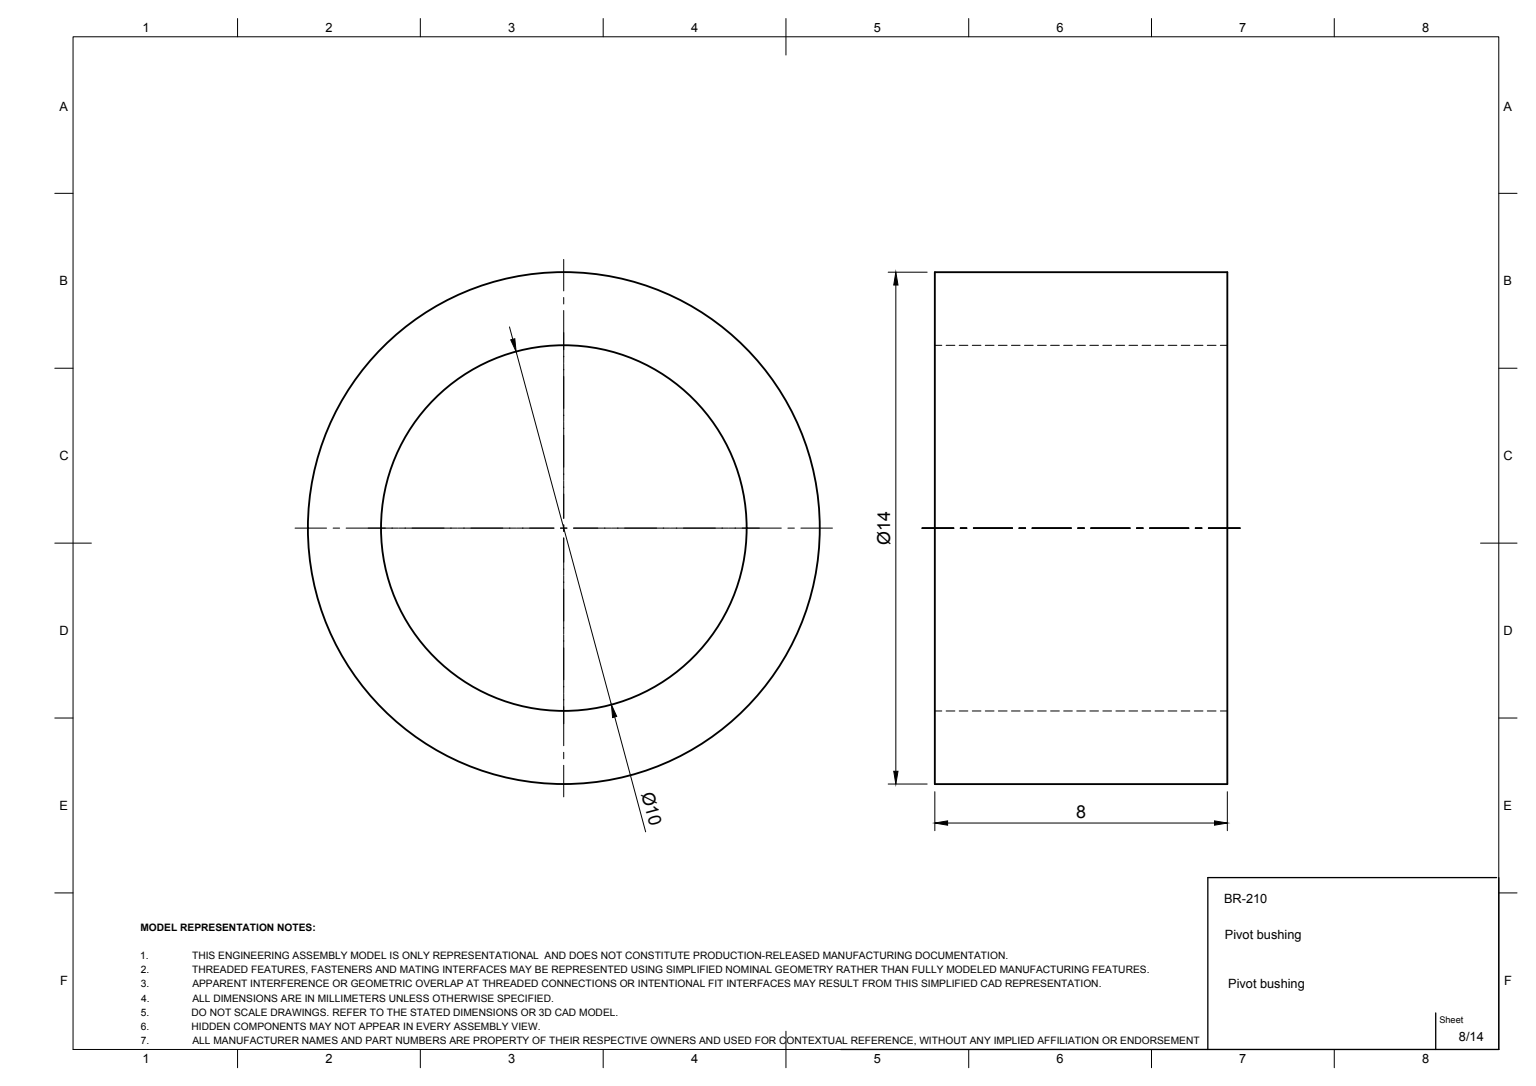
ISO-10303-21;
HEADER;
/* Generated by software containing ST-Developer
 * from STEP Tools, Inc. (www.steptools.com) 
 */

FILE_DESCRIPTION(
/* description */ ('Independent 1:2 reduction pantograph. 120 mm parallelogram sides; fix
ed fulcrum on the extension of a 240 mm link. Drawing point halfway al
ong its link, so its XY displacement is one half of the tracing point.
 Replaceable pivot bushes and retained pins. Calibration and productio
n accuracy unassigned.'),
/* implementation_level */ '2;1');

FILE_NAME(
/* name */ 'Pivot bushing.step',
/* time_stamp */ '2026-11-07T22:11:57-08:00',
/* author */ (''),
/* organization */ (''),
/* preprocessor_version */ 'ST-DEVELOPER v20.2',
/* originating_system */ 'Autodesk Translation Framework v15.17.0.0',
/* authorisation */ '');

FILE_SCHEMA (('AUTOMOTIVE_DESIGN { 1 0 10303 214 3 1 1 }'));
ENDSEC;

DATA;
#10=MECHANICAL_DESIGN_GEOMETRIC_PRESENTATION_REPRESENTATION('',(#194),#2926);
#168=SHAPE_REPRESENTATION_RELATIONSHIP('SRR','None',#3005,#181);
#181=ADVANCED_BREP_SHAPE_REPRESENTATION('',(#207),#2921);
#194=STYLED_ITEM('',(#3078),#207);
#207=MANIFOLD_SOLID_BREP('Body1',#1549);
#251=FACE_BOUND('',#505,.T.);
#252=FACE_BOUND('',#507,.T.);
#291=PLANE('',#1846);
#292=PLANE('',#1847);
#371=FACE_OUTER_BOUND('',#502,.T.);
#372=FACE_OUTER_BOUND('',#503,.T.);
#373=FACE_OUTER_BOUND('',#504,.T.);
#374=FACE_OUTER_BOUND('',#506,.T.);
#502=EDGE_LOOP('',(#1325,#1326,#1327,#1328));
#503=EDGE_LOOP('',(#1329,#1330,#1331,#1332));
#504=EDGE_LOOP('',(#1333));
#505=EDGE_LOOP('',(#1334));
#506=EDGE_LOOP('',(#1335));
#507=EDGE_LOOP('',(#1336));
#598=LINE('',#2767,#679);
#599=LINE('',#2773,#680);
#679=VECTOR('',#2280,5.);
#680=VECTOR('',#2287,7.);
#763=CIRCLE('',#1841,5.);
#764=CIRCLE('',#1842,5.);
#765=CIRCLE('',#1844,7.);
#766=CIRCLE('',#1845,7.);
#871=VERTEX_POINT('',#2764);
#872=VERTEX_POINT('',#2766);
#873=VERTEX_POINT('',#2770);
#874=VERTEX_POINT('',#2772);
#1027=EDGE_CURVE('',#871,#871,#763,.T.);
#1028=EDGE_CURVE('',#871,#872,#598,.T.);
#1029=EDGE_CURVE('',#872,#872,#764,.T.);
#1030=EDGE_CURVE('',#873,#873,#765,.T.);
#1031=EDGE_CURVE('',#873,#874,#599,.T.);
#1032=EDGE_CURVE('',#874,#874,#766,.T.);
#1325=ORIENTED_EDGE('',*,*,#1027,.F.);
#1326=ORIENTED_EDGE('',*,*,#1028,.T.);
#1327=ORIENTED_EDGE('',*,*,#1029,.T.);
#1328=ORIENTED_EDGE('',*,*,#1028,.F.);
#1329=ORIENTED_EDGE('',*,*,#1030,.F.);
#1330=ORIENTED_EDGE('',*,*,#1031,.T.);
#1331=ORIENTED_EDGE('',*,*,#1032,.T.);
#1332=ORIENTED_EDGE('',*,*,#1031,.F.);
#1333=ORIENTED_EDGE('',*,*,#1030,.T.);
#1334=ORIENTED_EDGE('',*,*,#1027,.T.);
#1335=ORIENTED_EDGE('',*,*,#1032,.F.);
#1336=ORIENTED_EDGE('',*,*,#1029,.F.);
#1438=CYLINDRICAL_SURFACE('',#1840,5.);
#1439=CYLINDRICAL_SURFACE('',#1843,7.);
#1515=ADVANCED_FACE('',(#371),#1438,.F.);
#1516=ADVANCED_FACE('',(#372),#1439,.T.);
#1517=ADVANCED_FACE('',(#373,#251),#291,.T.);
#1518=ADVANCED_FACE('',(#374,#252),#292,.F.);
#1549=CLOSED_SHELL('',(#1515,#1516,#1517,#1518));
#1839=AXIS2_PLACEMENT_3D('',#2762,#2274,#2275);
#1840=AXIS2_PLACEMENT_3D('',#2763,#2276,#2277);
#1841=AXIS2_PLACEMENT_3D('',#2765,#2278,#2279);
#1842=AXIS2_PLACEMENT_3D('',#2768,#2281,#2282);
#1843=AXIS2_PLACEMENT_3D('',#2769,#2283,#2284);
#1844=AXIS2_PLACEMENT_3D('',#2771,#2285,#2286);
#1845=AXIS2_PLACEMENT_3D('',#2774,#2288,#2289);
#1846=AXIS2_PLACEMENT_3D('',#2775,#2290,#2291);
#1847=AXIS2_PLACEMENT_3D('',#2776,#2292,#2293);
#2274=DIRECTION('axis',(0.,0.,1.));
#2275=DIRECTION('refdir',(1.,0.,0.));
#2276=DIRECTION('center_axis',(0.,0.,1.));
#2277=DIRECTION('ref_axis',(1.,0.,0.));
#2278=DIRECTION('center_axis',(0.,0.,-1.));
#2279=DIRECTION('ref_axis',(1.,0.,0.));
#2280=DIRECTION('',(0.,0.,-1.));
#2281=DIRECTION('center_axis',(0.,0.,-1.));
#2282=DIRECTION('ref_axis',(1.,0.,0.));
#2283=DIRECTION('center_axis',(0.,0.,1.));
#2284=DIRECTION('ref_axis',(1.,0.,0.));
#2285=DIRECTION('center_axis',(0.,0.,1.));
#2286=DIRECTION('ref_axis',(1.,0.,0.));
#2287=DIRECTION('',(0.,0.,-1.));
#2288=DIRECTION('center_axis',(0.,0.,1.));
#2289=DIRECTION('ref_axis',(1.,0.,0.));
#2290=DIRECTION('center_axis',(0.,0.,1.));
#2291=DIRECTION('ref_axis',(1.,0.,0.));
#2292=DIRECTION('center_axis',(0.,0.,1.));
#2293=DIRECTION('ref_axis',(1.,0.,0.));
#2762=CARTESIAN_POINT('',(0.,0.,0.));
#2763=CARTESIAN_POINT('Origin',(0.,0.,0.));
#2764=CARTESIAN_POINT('',(-5.,-6.12323399573677E-16,8.));
#2765=CARTESIAN_POINT('Origin',(0.,0.,8.));
#2766=CARTESIAN_POINT('',(-5.,-6.12323399573677E-16,0.));
#2767=CARTESIAN_POINT('',(-5.,-6.12323399573677E-16,0.));
#2768=CARTESIAN_POINT('Origin',(0.,0.,0.));
#2769=CARTESIAN_POINT('Origin',(0.,0.,0.));
#2770=CARTESIAN_POINT('',(-7.,-8.57252759403147E-16,8.));
#2771=CARTESIAN_POINT('Origin',(0.,0.,8.));
#2772=CARTESIAN_POINT('',(-7.,-8.57252759403147E-16,0.));
#2773=CARTESIAN_POINT('',(-7.,-8.57252759403147E-16,0.));
#2774=CARTESIAN_POINT('Origin',(0.,0.,0.));
#2775=CARTESIAN_POINT('Origin',(0.,0.,8.));
#2776=CARTESIAN_POINT('Origin',(0.,0.,0.));
#2906=UNCERTAINTY_MEASURE_WITH_UNIT(LENGTH_MEASURE(0.01),#2927,
'DISTANCE_ACCURACY_VALUE',
'Maximum model space distance between geometric entities at asserted c
onnectivities');
#2911=UNCERTAINTY_MEASURE_WITH_UNIT(LENGTH_MEASURE(0.01),#2927,
'DISTANCE_ACCURACY_VALUE',
'Maximum model space distance between geometric entities at asserted c
onnectivities');
#2921=(
GEOMETRIC_REPRESENTATION_CONTEXT(3)
GLOBAL_UNCERTAINTY_ASSIGNED_CONTEXT((#2906))
GLOBAL_UNIT_ASSIGNED_CONTEXT((#2927,#2929,#2930))
REPRESENTATION_CONTEXT('','3D')
);
#2926=(
GEOMETRIC_REPRESENTATION_CONTEXT(3)
GLOBAL_UNCERTAINTY_ASSIGNED_CONTEXT((#2911))
GLOBAL_UNIT_ASSIGNED_CONTEXT((#2927,#2929,#2930))
REPRESENTATION_CONTEXT('','3D')
);
#2927=(
LENGTH_UNIT()
NAMED_UNIT(*)
SI_UNIT(.MILLI.,.METRE.)
);
#2929=(
NAMED_UNIT(*)
PLANE_ANGLE_UNIT()
SI_UNIT($,.RADIAN.)
);
#2930=(
NAMED_UNIT(*)
SI_UNIT($,.STERADIAN.)
SOLID_ANGLE_UNIT()
);
#2940=SHAPE_DEFINITION_REPRESENTATION(#2954,#3005);
#2954=PRODUCT_DEFINITION_SHAPE('',$,#3020);
#3005=SHAPE_REPRESENTATION('',(#1839),#2921);
#3010=PRODUCT_DEFINITION_CONTEXT('part definition',#3054,'design');
#3020=PRODUCT_DEFINITION('Pivot bushing','Pivot bushing',#3034,#3010);
#3034=PRODUCT_DEFINITION_FORMATION('',$,#3065);
#3054=APPLICATION_CONTEXT(
'Core Data for Automotive Mechanical Design Process');
#3055=PRODUCT_CONTEXT('part definition',#3054,'mechanical');
#3065=PRODUCT('Pivot bushing','Pivot bushing',$,(#3055));
#3078=PRESENTATION_STYLE_ASSIGNMENT((#3090));
#3090=SURFACE_STYLE_USAGE(.BOTH.,#3102);
#3102=SURFACE_SIDE_STYLE('',(#3114));
#3114=SURFACE_STYLE_FILL_AREA(#3126);
#3126=FILL_AREA_STYLE('Bearing light gray',(#3138));
#3138=FILL_AREA_STYLE_COLOUR('Bearing light gray',#3150);
#3150=COLOUR_RGB('Bearing light gray',0.725490196078431,0.752941176470588,
0.792156862745098);
ENDSEC;
END-ISO-10303-21;
